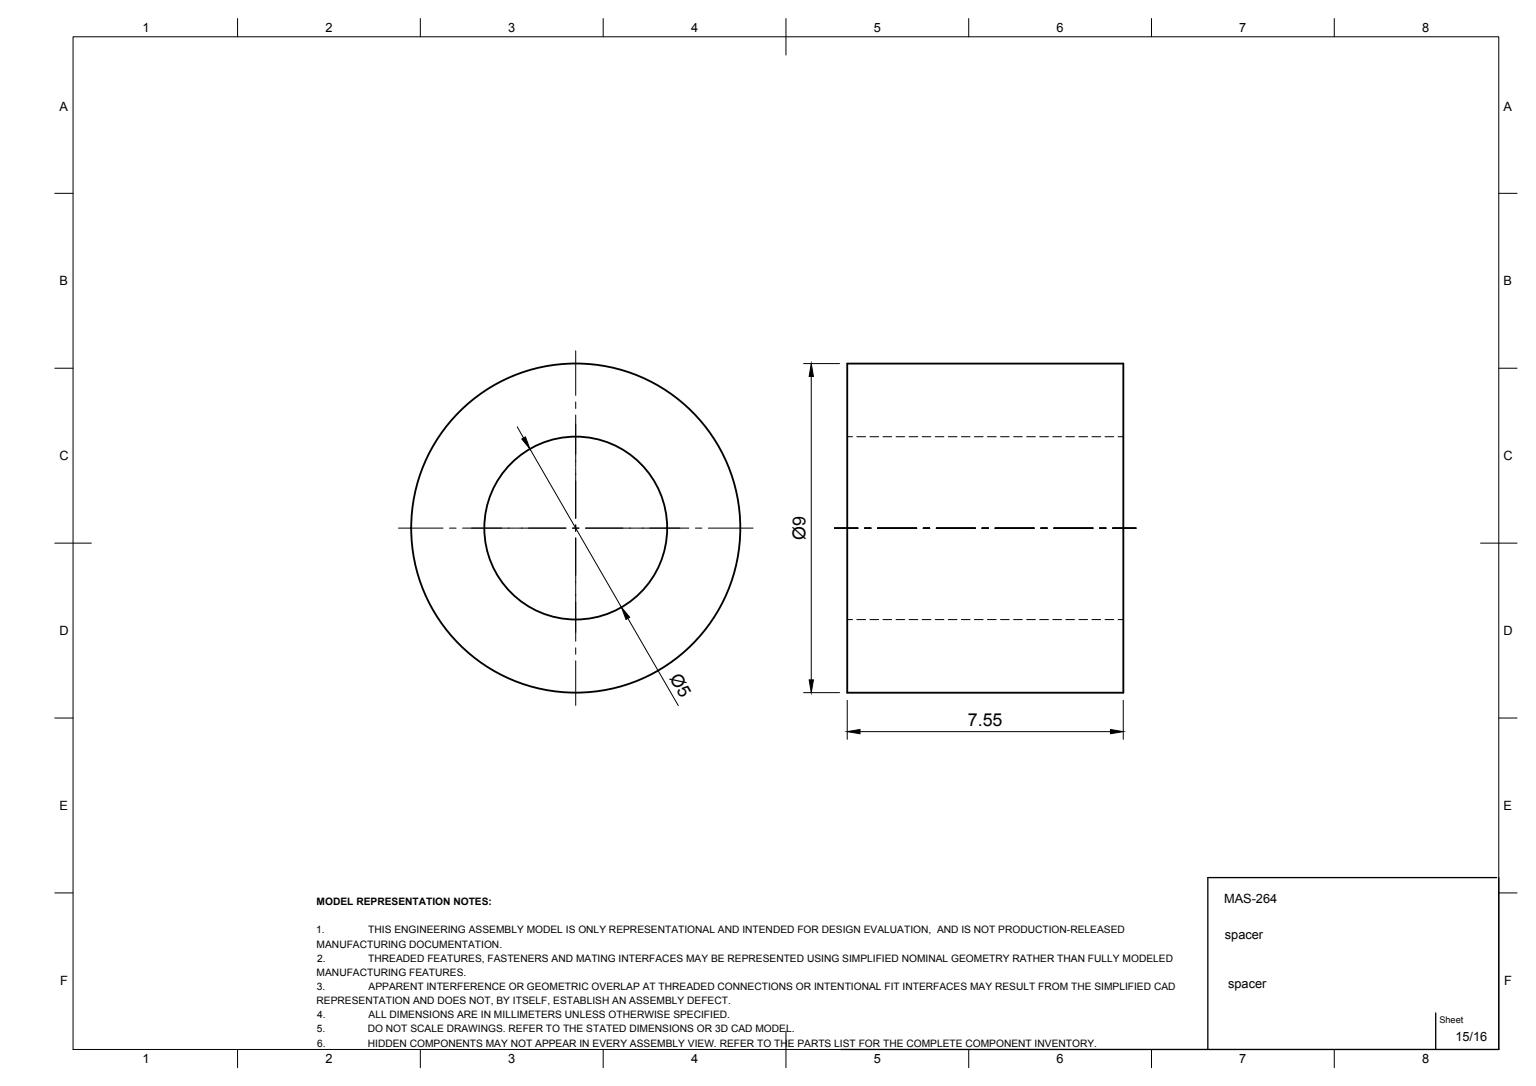
ISO-10303-21;
HEADER;
/* Generated by software containing ST-Developer
 * from STEP Tools, Inc. (www.steptools.com) 
 */

FILE_DESCRIPTION(
/* description */ (''),
/* implementation_level */ '2;1');

FILE_NAME(
/* name */ 'Spacer.step',
/* time_stamp */ '2026-10-12T15:37:13-07:00',
/* author */ (''),
/* organization */ (''),
/* preprocessor_version */ 'ST-DEVELOPER v20.2',
/* originating_system */ 'Autodesk Translation Framework v15.15.0.0',
/* authorisation */ '');

FILE_SCHEMA (('AUTOMOTIVE_DESIGN { 1 0 10303 214 3 1 1 }'));
ENDSEC;

DATA;
#10=MECHANICAL_DESIGN_GEOMETRIC_PRESENTATION_REPRESENTATION('',(#335),#36460);
#108=SHAPE_REPRESENTATION_RELATIONSHIP('SRR','None',#36520,#121);
#121=ADVANCED_BREP_SHAPE_REPRESENTATION('',(#367),#36449);
#161=FACE_BOUND('',#1984,.T.);
#162=FACE_BOUND('',#1986,.T.);
#335=STYLED_ITEM('',(#36598),#367);
#367=MANIFOLD_SOLID_BREP('Body1',#11271);
#523=PLANE('',#11908);
#524=PLANE('',#11909);
#1338=FACE_OUTER_BOUND('',#1981,.T.);
#1339=FACE_OUTER_BOUND('',#1982,.T.);
#1340=FACE_OUTER_BOUND('',#1983,.T.);
#1341=FACE_OUTER_BOUND('',#1985,.T.);
#1981=EDGE_LOOP('',(#8870,#8871,#8872,#8873));
#1982=EDGE_LOOP('',(#8874,#8875,#8876,#8877));
#1983=EDGE_LOOP('',(#8878));
#1984=EDGE_LOOP('',(#8879));
#1985=EDGE_LOOP('',(#8880));
#1986=EDGE_LOOP('',(#8881));
#2785=LINE('',#34642,#3731);
#2786=LINE('',#34648,#3732);
#3731=VECTOR('',#13766,2.5);
#3732=VECTOR('',#13773,4.49999999999999);
#4392=CIRCLE('',#11903,2.5);
#4393=CIRCLE('',#11904,2.5);
#4394=CIRCLE('',#11906,4.49999999999999);
#4395=CIRCLE('',#11907,4.49999999999999);
#5129=VERTEX_POINT('',#34639);
#5130=VERTEX_POINT('',#34641);
#5131=VERTEX_POINT('',#34645);
#5132=VERTEX_POINT('',#34647);
#6466=EDGE_CURVE('',#5129,#5129,#4392,.T.);
#6467=EDGE_CURVE('',#5129,#5130,#2785,.T.);
#6468=EDGE_CURVE('',#5130,#5130,#4393,.T.);
#6469=EDGE_CURVE('',#5131,#5131,#4394,.T.);
#6470=EDGE_CURVE('',#5131,#5132,#2786,.T.);
#6471=EDGE_CURVE('',#5132,#5132,#4395,.T.);
#8870=ORIENTED_EDGE('',*,*,#6466,.T.);
#8871=ORIENTED_EDGE('',*,*,#6467,.T.);
#8872=ORIENTED_EDGE('',*,*,#6468,.F.);
#8873=ORIENTED_EDGE('',*,*,#6467,.F.);
#8874=ORIENTED_EDGE('',*,*,#6469,.F.);
#8875=ORIENTED_EDGE('',*,*,#6470,.T.);
#8876=ORIENTED_EDGE('',*,*,#6471,.T.);
#8877=ORIENTED_EDGE('',*,*,#6470,.F.);
#8878=ORIENTED_EDGE('',*,*,#6469,.T.);
#8879=ORIENTED_EDGE('',*,*,#6468,.T.);
#8880=ORIENTED_EDGE('',*,*,#6471,.F.);
#8881=ORIENTED_EDGE('',*,*,#6466,.F.);
#10562=CYLINDRICAL_SURFACE('',#11902,2.5);
#10563=CYLINDRICAL_SURFACE('',#11905,4.49999999999999);
#10959=ADVANCED_FACE('',(#1338),#10562,.F.);
#10960=ADVANCED_FACE('',(#1339),#10563,.T.);
#10961=ADVANCED_FACE('',(#1340,#161),#523,.T.);
#10962=ADVANCED_FACE('',(#1341,#162),#524,.F.);
#11271=CLOSED_SHELL('',(#10959,#10960,#10961,#10962));
#11901=AXIS2_PLACEMENT_3D('',#34637,#13760,#13761);
#11902=AXIS2_PLACEMENT_3D('',#34638,#13762,#13763);
#11903=AXIS2_PLACEMENT_3D('',#34640,#13764,#13765);
#11904=AXIS2_PLACEMENT_3D('',#34643,#13767,#13768);
#11905=AXIS2_PLACEMENT_3D('',#34644,#13769,#13770);
#11906=AXIS2_PLACEMENT_3D('',#34646,#13771,#13772);
#11907=AXIS2_PLACEMENT_3D('',#34649,#13774,#13775);
#11908=AXIS2_PLACEMENT_3D('',#34650,#13776,#13777);
#11909=AXIS2_PLACEMENT_3D('',#34651,#13778,#13779);
#13760=DIRECTION('axis',(0.,0.,1.));
#13761=DIRECTION('refdir',(1.,0.,0.));
#13762=DIRECTION('center_axis',(1.,0.,0.));
#13763=DIRECTION('ref_axis',(0.,1.,0.));
#13764=DIRECTION('center_axis',(-1.,0.,0.));
#13765=DIRECTION('ref_axis',(0.,1.,0.));
#13766=DIRECTION('',(1.,0.,0.));
#13767=DIRECTION('center_axis',(-1.,0.,0.));
#13768=DIRECTION('ref_axis',(0.,1.,0.));
#13769=DIRECTION('center_axis',(1.,0.,0.));
#13770=DIRECTION('ref_axis',(0.,1.,0.));
#13771=DIRECTION('center_axis',(1.,0.,0.));
#13772=DIRECTION('ref_axis',(0.,1.,0.));
#13773=DIRECTION('',(-1.,0.,0.));
#13774=DIRECTION('center_axis',(1.,0.,0.));
#13775=DIRECTION('ref_axis',(0.,1.,0.));
#13776=DIRECTION('center_axis',(1.,0.,0.));
#13777=DIRECTION('ref_axis',(0.,1.,0.));
#13778=DIRECTION('center_axis',(1.,0.,0.));
#13779=DIRECTION('ref_axis',(0.,1.,0.));
#34637=CARTESIAN_POINT('',(0.,0.,0.));
#34638=CARTESIAN_POINT('Origin',(-22.5,190.828431883169,20.8299327490105));
#34639=CARTESIAN_POINT('',(-22.5,188.328431883169,20.8299327490105));
#34640=CARTESIAN_POINT('Origin',(-22.5,190.828431883169,20.8299327490105));
#34641=CARTESIAN_POINT('',(-14.95,188.328431883169,20.8299327490105));
#34642=CARTESIAN_POINT('',(-22.5,188.328431883169,20.8299327490105));
#34643=CARTESIAN_POINT('Origin',(-14.95,190.828431883169,20.8299327490105));
#34644=CARTESIAN_POINT('Origin',(-22.5,190.828431883169,20.8299327490105));
#34645=CARTESIAN_POINT('',(-14.95,186.328431883169,20.8299327490105));
#34646=CARTESIAN_POINT('Origin',(-14.95,190.828431883169,20.8299327490105));
#34647=CARTESIAN_POINT('',(-22.5,186.328431883169,20.8299327490105));
#34648=CARTESIAN_POINT('',(-22.5,186.328431883169,20.8299327490105));
#34649=CARTESIAN_POINT('Origin',(-22.5,190.828431883169,20.8299327490105));
#34650=CARTESIAN_POINT('Origin',(-14.95,190.828431883169,20.8299327490105));
#34651=CARTESIAN_POINT('Origin',(-22.5,190.828431883169,20.8299327490105));
#36433=UNCERTAINTY_MEASURE_WITH_UNIT(LENGTH_MEASURE(0.01),#36461,
'DISTANCE_ACCURACY_VALUE',
'Maximum model space distance between geometric entities at asserted c
onnectivities');
#36444=UNCERTAINTY_MEASURE_WITH_UNIT(LENGTH_MEASURE(0.01),#36461,
'DISTANCE_ACCURACY_VALUE',
'Maximum model space distance between geometric entities at asserted c
onnectivities');
#36449=(
GEOMETRIC_REPRESENTATION_CONTEXT(3)
GLOBAL_UNCERTAINTY_ASSIGNED_CONTEXT((#36433))
GLOBAL_UNIT_ASSIGNED_CONTEXT((#36461,#36463,#36464))
REPRESENTATION_CONTEXT('','3D')
);
#36460=(
GEOMETRIC_REPRESENTATION_CONTEXT(3)
GLOBAL_UNCERTAINTY_ASSIGNED_CONTEXT((#36444))
GLOBAL_UNIT_ASSIGNED_CONTEXT((#36461,#36463,#36464))
REPRESENTATION_CONTEXT('','3D')
);
#36461=(
LENGTH_UNIT()
NAMED_UNIT(*)
SI_UNIT(.MILLI.,.METRE.)
);
#36463=(
NAMED_UNIT(*)
PLANE_ANGLE_UNIT()
SI_UNIT($,.RADIAN.)
);
#36464=(
NAMED_UNIT(*)
SI_UNIT($,.STERADIAN.)
SOLID_ANGLE_UNIT()
);
#36469=SHAPE_DEFINITION_REPRESENTATION(#36484,#36520);
#36484=PRODUCT_DEFINITION_SHAPE('',$,#36536);
#36520=SHAPE_REPRESENTATION('',(#11901),#36449);
#36531=PRODUCT_DEFINITION_CONTEXT('part definition',#36578,'design');
#36536=PRODUCT_DEFINITION('spacer','Spacer',#36551,#36531);
#36551=PRODUCT_DEFINITION_FORMATION('',$,#36584);
#36578=APPLICATION_CONTEXT(
'Core Data for Automotive Mechanical Design Process');
#36579=PRODUCT_CONTEXT('part definition',#36578,'mechanical');
#36584=PRODUCT('spacer','Spacer',$,(#36579));
#36598=PRESENTATION_STYLE_ASSIGNMENT((#36603));
#36603=SURFACE_STYLE_USAGE(.BOTH.,#36608);
#36608=SURFACE_SIDE_STYLE('',(#36613));
#36613=SURFACE_STYLE_FILL_AREA(#36618);
#36618=FILL_AREA_STYLE('Opaque(245,245,246)',(#36623));
#36623=FILL_AREA_STYLE_COLOUR('Opaque(245,245,246)',#36628);
#36628=COLOUR_RGB('Opaque(245,245,246)', 0.40784314, 0.44705882, 0.49803922);
ENDSEC;
END-ISO-10303-21;
